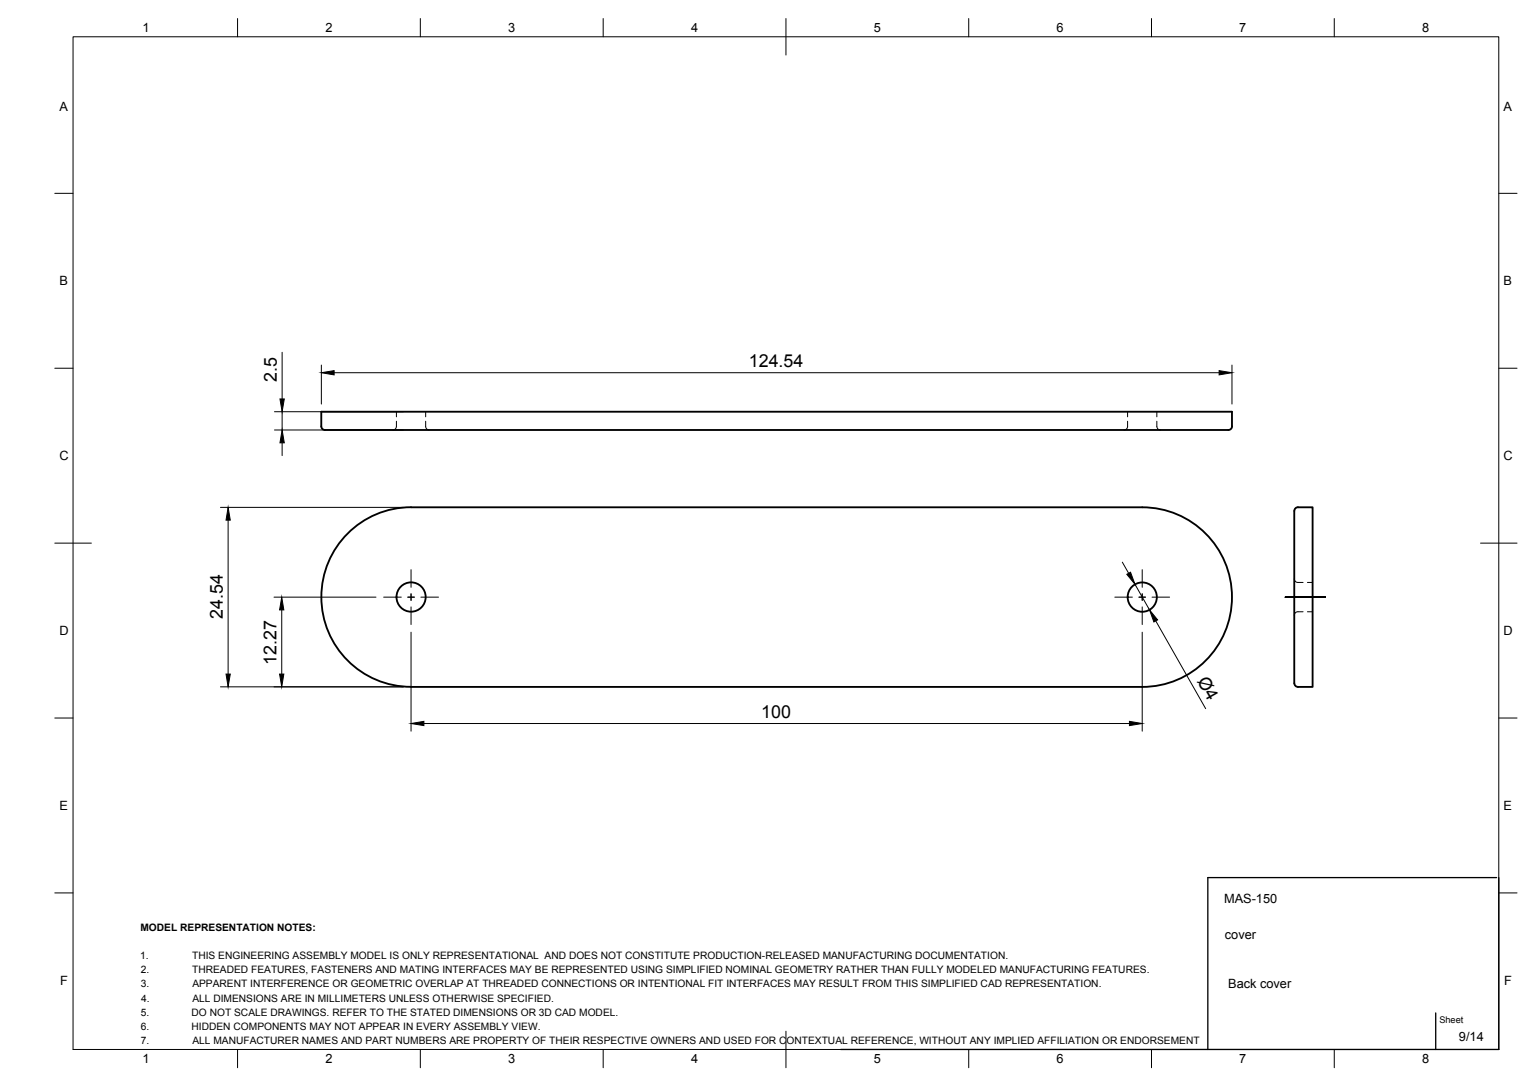
ISO-10303-21;
HEADER;
/* Generated by software containing ST-Developer
 * from STEP Tools, Inc. (www.steptools.com) 
 */

FILE_DESCRIPTION(
/* description */ ('STEP AP203'),
/* implementation_level */ '2;1');

FILE_NAME(
/* name */ 'Back cover.step',
/* time_stamp */ '2026-11-08T21:40:52-08:00',
/* author */ (''),
/* organization */ (''),
/* preprocessor_version */ 'ST-DEVELOPER v20.2',
/* originating_system */ 'Autodesk Translation Framework v15.17.0.0',
/* authorisation */ '');

FILE_SCHEMA (('AUTOMOTIVE_DESIGN { 1 0 10303 214 3 1 1 }'));
ENDSEC;

DATA;
#10=MECHANICAL_DESIGN_GEOMETRIC_PRESENTATION_REPRESENTATION('',(#191),#12137);
#169=SHAPE_REPRESENTATION_RELATIONSHIP('SRR','None',#12193,#180);
#180=ADVANCED_BREP_SHAPE_REPRESENTATION('',(#202),#12134);
#191=STYLED_ITEM('',(#12253),#202);
#202=MANIFOLD_SOLID_BREP('Body1',#1836);
#223=FACE_BOUND('',#704,.T.);
#224=FACE_BOUND('',#705,.T.);
#225=FACE_BOUND('',#707,.T.);
#226=FACE_BOUND('',#708,.T.);
#265=PLANE('',#2095);
#266=PLANE('',#2098);
#267=PLANE('',#2103);
#268=PLANE('',#2106);
#346=LINE('',#11987,#440);
#347=LINE('',#11991,#441);
#348=LINE('',#11998,#442);
#349=LINE('',#12001,#443);
#350=LINE('',#12007,#444);
#351=LINE('',#12010,#445);
#352=LINE('',#12013,#446);
#353=LINE('',#12016,#447);
#354=LINE('',#12019,#448);
#355=LINE('',#12020,#449);
#356=LINE('',#12023,#450);
#357=LINE('',#12026,#451);
#440=VECTOR('',#2492,2.);
#441=VECTOR('',#2497,2.);
#442=VECTOR('',#2504,1000.);
#443=VECTOR('',#2507,1000.);
#444=VECTOR('',#2512,1000.);
#445=VECTOR('',#2515,1000.);
#446=VECTOR('',#2518,1000.);
#447=VECTOR('',#2521,1000.);
#448=VECTOR('',#2524,1000.);
#449=VECTOR('',#2525,1000.);
#450=VECTOR('',#2528,1000.);
#451=VECTOR('',#2533,1000.);
#478=CYLINDRICAL_SURFACE('',#2091,2.);
#479=CYLINDRICAL_SURFACE('',#2093,2.);
#480=CYLINDRICAL_SURFACE('',#2101,12.2723008899906);
#481=CYLINDRICAL_SURFACE('',#2104,12.2723008899906);
#482=CYLINDRICAL_SURFACE('',#2107,0.5);
#483=CYLINDRICAL_SURFACE('',#2114,0.5);
#571=FACE_OUTER_BOUND('',#699,.T.);
#572=FACE_OUTER_BOUND('',#700,.T.);
#573=FACE_OUTER_BOUND('',#701,.T.);
#574=FACE_OUTER_BOUND('',#702,.T.);
#575=FACE_OUTER_BOUND('',#703,.T.);
#576=FACE_OUTER_BOUND('',#706,.T.);
#577=FACE_OUTER_BOUND('',#709,.T.);
#578=FACE_OUTER_BOUND('',#710,.T.);
#579=FACE_OUTER_BOUND('',#711,.T.);
#580=FACE_OUTER_BOUND('',#712,.T.);
#581=FACE_OUTER_BOUND('',#713,.T.);
#582=FACE_OUTER_BOUND('',#714,.T.);
#583=FACE_OUTER_BOUND('',#715,.T.);
#584=FACE_OUTER_BOUND('',#716,.T.);
#699=EDGE_LOOP('',(#1587,#1588,#1589,#1590,#1591));
#700=EDGE_LOOP('',(#1592,#1593,#1594,#1595,#1596));
#701=EDGE_LOOP('',(#1597,#1598,#1599,#1600,#1601));
#702=EDGE_LOOP('',(#1602,#1603,#1604,#1605,#1606));
#703=EDGE_LOOP('',(#1607,#1608,#1609,#1610));
#704=EDGE_LOOP('',(#1611));
#705=EDGE_LOOP('',(#1612));
#706=EDGE_LOOP('',(#1613,#1614,#1615,#1616));
#707=EDGE_LOOP('',(#1617));
#708=EDGE_LOOP('',(#1618));
#709=EDGE_LOOP('',(#1619,#1620,#1621,#1622));
#710=EDGE_LOOP('',(#1623,#1624,#1625,#1626));
#711=EDGE_LOOP('',(#1627,#1628,#1629,#1630));
#712=EDGE_LOOP('',(#1631,#1632,#1633,#1634));
#713=EDGE_LOOP('',(#1635,#1636,#1637,#1638));
#714=EDGE_LOOP('',(#1639,#1640,#1641,#1642));
#715=EDGE_LOOP('',(#1643,#1644,#1645,#1646));
#716=EDGE_LOOP('',(#1647,#1648,#1649,#1650));
#788=CIRCLE('',#2082,2.);
#789=CIRCLE('',#2083,2.);
#790=CIRCLE('',#2084,0.5);
#791=CIRCLE('',#2085,2.5);
#792=CIRCLE('',#2087,2.);
#793=CIRCLE('',#2088,2.);
#794=CIRCLE('',#2089,0.5);
#795=CIRCLE('',#2090,2.5);
#796=CIRCLE('',#2092,2.);
#797=CIRCLE('',#2094,2.);
#798=CIRCLE('',#2096,11.7723008899906);
#799=CIRCLE('',#2097,11.7723008899906);
#800=CIRCLE('',#2099,12.2723008899906);
#801=CIRCLE('',#2100,12.2723008899906);
#802=CIRCLE('',#2102,12.2723008899906);
#803=CIRCLE('',#2105,12.2723008899906);
#804=CIRCLE('',#2108,0.5);
#805=CIRCLE('',#2109,0.5);
#806=CIRCLE('',#2111,0.5);
#807=CIRCLE('',#2113,0.5);
#943=VERTEX_POINT('',#11970);
#944=VERTEX_POINT('',#11971);
#945=VERTEX_POINT('',#11974);
#946=VERTEX_POINT('',#11978);
#947=VERTEX_POINT('',#11979);
#948=VERTEX_POINT('',#11982);
#949=VERTEX_POINT('',#11986);
#950=VERTEX_POINT('',#11990);
#951=VERTEX_POINT('',#11994);
#952=VERTEX_POINT('',#11995);
#953=VERTEX_POINT('',#11997);
#954=VERTEX_POINT('',#11999);
#955=VERTEX_POINT('',#12003);
#956=VERTEX_POINT('',#12004);
#957=VERTEX_POINT('',#12006);
#958=VERTEX_POINT('',#12008);
#959=VERTEX_POINT('',#12012);
#960=VERTEX_POINT('',#12014);
#961=VERTEX_POINT('',#12018);
#962=VERTEX_POINT('',#12022);
#1163=EDGE_CURVE('',#943,#944,#788,.T.);
#1164=EDGE_CURVE('',#944,#943,#789,.T.);
#1165=EDGE_CURVE('',#944,#945,#790,.T.);
#1166=EDGE_CURVE('',#945,#945,#791,.T.);
#1167=EDGE_CURVE('',#946,#947,#792,.T.);
#1168=EDGE_CURVE('',#947,#946,#793,.T.);
#1169=EDGE_CURVE('',#947,#948,#794,.T.);
#1170=EDGE_CURVE('',#948,#948,#795,.T.);
#1171=EDGE_CURVE('',#946,#949,#346,.T.);
#1172=EDGE_CURVE('',#949,#949,#796,.T.);
#1173=EDGE_CURVE('',#943,#950,#347,.T.);
#1174=EDGE_CURVE('',#950,#950,#797,.T.);
#1175=EDGE_CURVE('',#951,#952,#798,.T.);
#1176=EDGE_CURVE('',#952,#953,#348,.T.);
#1177=EDGE_CURVE('',#953,#954,#799,.T.);
#1178=EDGE_CURVE('',#954,#951,#349,.T.);
#1179=EDGE_CURVE('',#955,#956,#800,.T.);
#1180=EDGE_CURVE('',#957,#955,#350,.T.);
#1181=EDGE_CURVE('',#958,#957,#801,.T.);
#1182=EDGE_CURVE('',#956,#958,#351,.T.);
#1183=EDGE_CURVE('',#959,#956,#352,.T.);
#1184=EDGE_CURVE('',#959,#960,#802,.T.);
#1185=EDGE_CURVE('',#960,#955,#353,.T.);
#1186=EDGE_CURVE('',#961,#958,#354,.T.);
#1187=EDGE_CURVE('',#961,#959,#355,.T.);
#1188=EDGE_CURVE('',#962,#957,#356,.T.);
#1189=EDGE_CURVE('',#962,#961,#803,.T.);
#1190=EDGE_CURVE('',#960,#962,#357,.T.);
#1191=EDGE_CURVE('',#959,#954,#804,.T.);
#1192=EDGE_CURVE('',#951,#961,#805,.T.);
#1193=EDGE_CURVE('',#952,#962,#806,.T.);
#1194=EDGE_CURVE('',#960,#953,#807,.T.);
#1587=ORIENTED_EDGE('',*,*,#1163,.F.);
#1588=ORIENTED_EDGE('',*,*,#1164,.F.);
#1589=ORIENTED_EDGE('',*,*,#1165,.T.);
#1590=ORIENTED_EDGE('',*,*,#1166,.F.);
#1591=ORIENTED_EDGE('',*,*,#1165,.F.);
#1592=ORIENTED_EDGE('',*,*,#1167,.F.);
#1593=ORIENTED_EDGE('',*,*,#1168,.F.);
#1594=ORIENTED_EDGE('',*,*,#1169,.T.);
#1595=ORIENTED_EDGE('',*,*,#1170,.F.);
#1596=ORIENTED_EDGE('',*,*,#1169,.F.);
#1597=ORIENTED_EDGE('',*,*,#1167,.T.);
#1598=ORIENTED_EDGE('',*,*,#1168,.T.);
#1599=ORIENTED_EDGE('',*,*,#1171,.T.);
#1600=ORIENTED_EDGE('',*,*,#1172,.F.);
#1601=ORIENTED_EDGE('',*,*,#1171,.F.);
#1602=ORIENTED_EDGE('',*,*,#1163,.T.);
#1603=ORIENTED_EDGE('',*,*,#1164,.T.);
#1604=ORIENTED_EDGE('',*,*,#1173,.T.);
#1605=ORIENTED_EDGE('',*,*,#1174,.F.);
#1606=ORIENTED_EDGE('',*,*,#1173,.F.);
#1607=ORIENTED_EDGE('',*,*,#1175,.T.);
#1608=ORIENTED_EDGE('',*,*,#1176,.T.);
#1609=ORIENTED_EDGE('',*,*,#1177,.T.);
#1610=ORIENTED_EDGE('',*,*,#1178,.T.);
#1611=ORIENTED_EDGE('',*,*,#1166,.T.);
#1612=ORIENTED_EDGE('',*,*,#1170,.T.);
#1613=ORIENTED_EDGE('',*,*,#1179,.F.);
#1614=ORIENTED_EDGE('',*,*,#1180,.F.);
#1615=ORIENTED_EDGE('',*,*,#1181,.F.);
#1616=ORIENTED_EDGE('',*,*,#1182,.F.);
#1617=ORIENTED_EDGE('',*,*,#1174,.T.);
#1618=ORIENTED_EDGE('',*,*,#1172,.T.);
#1619=ORIENTED_EDGE('',*,*,#1183,.F.);
#1620=ORIENTED_EDGE('',*,*,#1184,.T.);
#1621=ORIENTED_EDGE('',*,*,#1185,.T.);
#1622=ORIENTED_EDGE('',*,*,#1179,.T.);
#1623=ORIENTED_EDGE('',*,*,#1186,.F.);
#1624=ORIENTED_EDGE('',*,*,#1187,.T.);
#1625=ORIENTED_EDGE('',*,*,#1183,.T.);
#1626=ORIENTED_EDGE('',*,*,#1182,.T.);
#1627=ORIENTED_EDGE('',*,*,#1188,.F.);
#1628=ORIENTED_EDGE('',*,*,#1189,.T.);
#1629=ORIENTED_EDGE('',*,*,#1186,.T.);
#1630=ORIENTED_EDGE('',*,*,#1181,.T.);
#1631=ORIENTED_EDGE('',*,*,#1185,.F.);
#1632=ORIENTED_EDGE('',*,*,#1190,.T.);
#1633=ORIENTED_EDGE('',*,*,#1188,.T.);
#1634=ORIENTED_EDGE('',*,*,#1180,.T.);
#1635=ORIENTED_EDGE('',*,*,#1191,.F.);
#1636=ORIENTED_EDGE('',*,*,#1187,.F.);
#1637=ORIENTED_EDGE('',*,*,#1192,.F.);
#1638=ORIENTED_EDGE('',*,*,#1178,.F.);
#1639=ORIENTED_EDGE('',*,*,#1192,.T.);
#1640=ORIENTED_EDGE('',*,*,#1189,.F.);
#1641=ORIENTED_EDGE('',*,*,#1193,.F.);
#1642=ORIENTED_EDGE('',*,*,#1175,.F.);
#1643=ORIENTED_EDGE('',*,*,#1191,.T.);
#1644=ORIENTED_EDGE('',*,*,#1177,.F.);
#1645=ORIENTED_EDGE('',*,*,#1194,.F.);
#1646=ORIENTED_EDGE('',*,*,#1184,.F.);
#1647=ORIENTED_EDGE('',*,*,#1193,.T.);
#1648=ORIENTED_EDGE('',*,*,#1190,.F.);
#1649=ORIENTED_EDGE('',*,*,#1194,.T.);
#1650=ORIENTED_EDGE('',*,*,#1176,.F.);
#1712=TOROIDAL_SURFACE('',#2081,2.5,0.5);
#1713=TOROIDAL_SURFACE('',#2086,2.5,0.5);
#1714=TOROIDAL_SURFACE('',#2110,11.7723008899906,0.5);
#1715=TOROIDAL_SURFACE('',#2112,11.7723008899906,0.5);
#1799=ADVANCED_FACE('',(#571),#1712,.T.);
#1800=ADVANCED_FACE('',(#572),#1713,.T.);
#1801=ADVANCED_FACE('',(#573),#478,.F.);
#1802=ADVANCED_FACE('',(#574),#479,.F.);
#1803=ADVANCED_FACE('',(#575,#223,#224),#265,.T.);
#1804=ADVANCED_FACE('',(#576,#225,#226),#266,.F.);
#1805=ADVANCED_FACE('',(#577),#480,.T.);
#1806=ADVANCED_FACE('',(#578),#267,.F.);
#1807=ADVANCED_FACE('',(#579),#481,.T.);
#1808=ADVANCED_FACE('',(#580),#268,.F.);
#1809=ADVANCED_FACE('',(#581),#482,.T.);
#1810=ADVANCED_FACE('',(#582),#1714,.T.);
#1811=ADVANCED_FACE('',(#583),#1715,.T.);
#1812=ADVANCED_FACE('',(#584),#483,.T.);
#1836=CLOSED_SHELL('',(#1799,#1800,#1801,#1802,#1803,#1804,#1805,#1806,
#1807,#1808,#1809,#1810,#1811,#1812));
#2080=AXIS2_PLACEMENT_3D('',#11968,#2468,#2469);
#2081=AXIS2_PLACEMENT_3D('',#11969,#2470,#2471);
#2082=AXIS2_PLACEMENT_3D('',#11972,#2472,#2473);
#2083=AXIS2_PLACEMENT_3D('',#11973,#2474,#2475);
#2084=AXIS2_PLACEMENT_3D('',#11975,#2476,#2477);
#2085=AXIS2_PLACEMENT_3D('',#11976,#2478,#2479);
#2086=AXIS2_PLACEMENT_3D('',#11977,#2480,#2481);
#2087=AXIS2_PLACEMENT_3D('',#11980,#2482,#2483);
#2088=AXIS2_PLACEMENT_3D('',#11981,#2484,#2485);
#2089=AXIS2_PLACEMENT_3D('',#11983,#2486,#2487);
#2090=AXIS2_PLACEMENT_3D('',#11984,#2488,#2489);
#2091=AXIS2_PLACEMENT_3D('',#11985,#2490,#2491);
#2092=AXIS2_PLACEMENT_3D('',#11988,#2493,#2494);
#2093=AXIS2_PLACEMENT_3D('',#11989,#2495,#2496);
#2094=AXIS2_PLACEMENT_3D('',#11992,#2498,#2499);
#2095=AXIS2_PLACEMENT_3D('',#11993,#2500,#2501);
#2096=AXIS2_PLACEMENT_3D('',#11996,#2502,#2503);
#2097=AXIS2_PLACEMENT_3D('',#12000,#2505,#2506);
#2098=AXIS2_PLACEMENT_3D('',#12002,#2508,#2509);
#2099=AXIS2_PLACEMENT_3D('',#12005,#2510,#2511);
#2100=AXIS2_PLACEMENT_3D('',#12009,#2513,#2514);
#2101=AXIS2_PLACEMENT_3D('',#12011,#2516,#2517);
#2102=AXIS2_PLACEMENT_3D('',#12015,#2519,#2520);
#2103=AXIS2_PLACEMENT_3D('',#12017,#2522,#2523);
#2104=AXIS2_PLACEMENT_3D('',#12021,#2526,#2527);
#2105=AXIS2_PLACEMENT_3D('',#12024,#2529,#2530);
#2106=AXIS2_PLACEMENT_3D('',#12025,#2531,#2532);
#2107=AXIS2_PLACEMENT_3D('',#12027,#2534,#2535);
#2108=AXIS2_PLACEMENT_3D('',#12028,#2536,#2537);
#2109=AXIS2_PLACEMENT_3D('',#12029,#2538,#2539);
#2110=AXIS2_PLACEMENT_3D('',#12030,#2540,#2541);
#2111=AXIS2_PLACEMENT_3D('',#12031,#2542,#2543);
#2112=AXIS2_PLACEMENT_3D('',#12032,#2544,#2545);
#2113=AXIS2_PLACEMENT_3D('',#12033,#2546,#2547);
#2114=AXIS2_PLACEMENT_3D('',#12034,#2548,#2549);
#2468=DIRECTION('axis',(0.,0.,1.));
#2469=DIRECTION('refdir',(1.,0.,0.));
#2470=DIRECTION('center_axis',(0.,1.,0.));
#2471=DIRECTION('ref_axis',(0.,0.,1.));
#2472=DIRECTION('center_axis',(0.,1.,0.));
#2473=DIRECTION('ref_axis',(0.,0.,1.));
#2474=DIRECTION('center_axis',(0.,1.,0.));
#2475=DIRECTION('ref_axis',(0.,0.,1.));
#2476=DIRECTION('center_axis',(-1.,0.,0.));
#2477=DIRECTION('ref_axis',(0.,0.,-1.));
#2478=DIRECTION('center_axis',(0.,-1.,0.));
#2479=DIRECTION('ref_axis',(0.,0.,1.));
#2480=DIRECTION('center_axis',(0.,1.,0.));
#2481=DIRECTION('ref_axis',(0.,0.,1.));
#2482=DIRECTION('center_axis',(0.,1.,0.));
#2483=DIRECTION('ref_axis',(0.,0.,1.));
#2484=DIRECTION('center_axis',(0.,1.,0.));
#2485=DIRECTION('ref_axis',(0.,0.,1.));
#2486=DIRECTION('center_axis',(-1.,0.,0.));
#2487=DIRECTION('ref_axis',(0.,0.,-1.));
#2488=DIRECTION('center_axis',(0.,-1.,0.));
#2489=DIRECTION('ref_axis',(0.,0.,1.));
#2490=DIRECTION('center_axis',(0.,-1.,0.));
#2491=DIRECTION('ref_axis',(0.,0.,-1.));
#2492=DIRECTION('',(0.,-1.,0.));
#2493=DIRECTION('center_axis',(0.,1.,0.));
#2494=DIRECTION('ref_axis',(0.,0.,1.));
#2495=DIRECTION('center_axis',(0.,-1.,0.));
#2496=DIRECTION('ref_axis',(0.,0.,-1.));
#2497=DIRECTION('',(0.,-1.,0.));
#2498=DIRECTION('center_axis',(0.,1.,0.));
#2499=DIRECTION('ref_axis',(0.,0.,1.));
#2500=DIRECTION('center_axis',(0.,1.,0.));
#2501=DIRECTION('ref_axis',(0.,0.,1.));
#2502=DIRECTION('center_axis',(0.,1.,0.));
#2503=DIRECTION('ref_axis',(0.,0.,1.));
#2504=DIRECTION('',(1.,0.,-7.77156117237611E-15));
#2505=DIRECTION('center_axis',(0.,1.,0.));
#2506=DIRECTION('ref_axis',(0.,0.,1.));
#2507=DIRECTION('',(-1.,0.,7.77156117237609E-15));
#2508=DIRECTION('center_axis',(0.,1.,0.));
#2509=DIRECTION('ref_axis',(0.,0.,1.));
#2510=DIRECTION('center_axis',(0.,1.,0.));
#2511=DIRECTION('ref_axis',(0.,0.,1.));
#2512=DIRECTION('',(1.,0.,-7.77156117237611E-15));
#2513=DIRECTION('center_axis',(0.,1.,0.));
#2514=DIRECTION('ref_axis',(0.,0.,1.));
#2515=DIRECTION('',(-1.,0.,7.77156117237609E-15));
#2516=DIRECTION('center_axis',(0.,-1.,0.));
#2517=DIRECTION('ref_axis',(0.,0.,-1.));
#2518=DIRECTION('',(0.,-1.,0.));
#2519=DIRECTION('center_axis',(0.,-1.,0.));
#2520=DIRECTION('ref_axis',(0.,0.,1.));
#2521=DIRECTION('',(0.,-1.,0.));
#2522=DIRECTION('center_axis',(7.77156117237609E-15,0.,1.));
#2523=DIRECTION('ref_axis',(1.,0.,-7.77156117237609E-15));
#2524=DIRECTION('',(0.,-1.,0.));
#2525=DIRECTION('',(1.,0.,-7.77156117237609E-15));
#2526=DIRECTION('center_axis',(0.,-1.,0.));
#2527=DIRECTION('ref_axis',(0.,0.,-1.));
#2528=DIRECTION('',(0.,-1.,0.));
#2529=DIRECTION('center_axis',(0.,-1.,0.));
#2530=DIRECTION('ref_axis',(0.,0.,1.));
#2531=DIRECTION('center_axis',(-7.77156117237611E-15,0.,-1.));
#2532=DIRECTION('ref_axis',(-1.,0.,7.77156117237611E-15));
#2533=DIRECTION('',(-1.,0.,7.77156117237611E-15));
#2534=DIRECTION('center_axis',(1.,0.,-7.77156117237609E-15));
#2535=DIRECTION('ref_axis',(-7.77156117237609E-15,0.,-1.));
#2536=DIRECTION('center_axis',(1.,0.,-6.93889390390722E-15));
#2537=DIRECTION('ref_axis',(-6.93889390390722E-15,0.,-1.));
#2538=DIRECTION('center_axis',(-1.,0.,0.));
#2539=DIRECTION('ref_axis',(0.,0.,1.));
#2540=DIRECTION('center_axis',(0.,1.,0.));
#2541=DIRECTION('ref_axis',(0.,0.,1.));
#2542=DIRECTION('center_axis',(1.,0.,0.));
#2543=DIRECTION('ref_axis',(0.,0.,-1.));
#2544=DIRECTION('center_axis',(0.,1.,0.));
#2545=DIRECTION('ref_axis',(0.,0.,1.));
#2546=DIRECTION('center_axis',(-1.,-6.93889390390723E-15,0.));
#2547=DIRECTION('ref_axis',(6.93889390390723E-15,-1.,0.));
#2548=DIRECTION('center_axis',(-1.,0.,7.77156117237611E-15));
#2549=DIRECTION('ref_axis',(7.77156117237611E-15,0.,1.));
#11968=CARTESIAN_POINT('',(0.,0.,0.));
#11969=CARTESIAN_POINT('Origin',(-83.4892602927113,2.,28.6344795489034));
#11970=CARTESIAN_POINT('',(-83.4892602927113,2.,30.6344795489034));
#11971=CARTESIAN_POINT('',(-83.4892602927113,2.,26.6344795489034));
#11972=CARTESIAN_POINT('Origin',(-83.4892602927113,2.,28.6344795489034));
#11973=CARTESIAN_POINT('Origin',(-83.4892602927113,2.,28.6344795489034));
#11974=CARTESIAN_POINT('',(-83.4892602927113,2.5,26.1344795489034));
#11975=CARTESIAN_POINT('Origin',(-83.4892602927113,2.,26.1344795489034));
#11976=CARTESIAN_POINT('Origin',(-83.4892602927113,2.5,28.6344795489034));
#11977=CARTESIAN_POINT('Origin',(16.5107397072887,2.,28.6344795489026));
#11978=CARTESIAN_POINT('',(16.5107397072887,2.,30.6344795489026));
#11979=CARTESIAN_POINT('',(16.5107397072887,2.,26.6344795489026));
#11980=CARTESIAN_POINT('Origin',(16.5107397072887,2.,28.6344795489026));
#11981=CARTESIAN_POINT('Origin',(16.5107397072887,2.,28.6344795489026));
#11982=CARTESIAN_POINT('',(16.5107397072887,2.5,26.1344795489026));
#11983=CARTESIAN_POINT('Origin',(16.5107397072887,2.,26.1344795489026));
#11984=CARTESIAN_POINT('Origin',(16.5107397072887,2.5,28.6344795489026));
#11985=CARTESIAN_POINT('Origin',(16.5107397072887,2.5,28.6344795489026));
#11986=CARTESIAN_POINT('',(16.5107397072887,0.,30.6344795489026));
#11987=CARTESIAN_POINT('',(16.5107397072887,2.5,30.6344795489026));
#11988=CARTESIAN_POINT('Origin',(16.5107397072887,0.,28.6344795489026));
#11989=CARTESIAN_POINT('Origin',(-83.4892602927113,2.5,28.6344795489034));
#11990=CARTESIAN_POINT('',(-83.4892602927113,0.,30.6344795489034));
#11991=CARTESIAN_POINT('',(-83.4892602927113,2.5,30.6344795489034));
#11992=CARTESIAN_POINT('Origin',(-83.4892602927113,0.,28.6344795489034));
#11993=CARTESIAN_POINT('Origin',(16.5107397072887,2.5,28.6344795489026));
#11994=CARTESIAN_POINT('',(-83.4892602927114,2.49999999999999,16.8621786589128));
#11995=CARTESIAN_POINT('',(-83.4892602927112,2.5,40.406780438894));
#11996=CARTESIAN_POINT('Origin',(-83.4892602927113,2.5,28.6344795489034));
#11997=CARTESIAN_POINT('',(16.5107397072887,2.5,40.4067804388932));
#11998=CARTESIAN_POINT('',(16.5107397072887,2.5,40.4067804388932));
#11999=CARTESIAN_POINT('',(16.5107397072887,2.49999999999999,16.862178658912));
#12000=CARTESIAN_POINT('Origin',(16.5107397072887,2.5,28.6344795489026));
#12001=CARTESIAN_POINT('',(-83.4892602927114,2.49999999999999,16.8621786589128));
#12002=CARTESIAN_POINT('Origin',(16.5107397072887,0.,28.6344795489026));
#12003=CARTESIAN_POINT('',(16.5107397072887,-1.38777878078145E-14,40.9067804388932));
#12004=CARTESIAN_POINT('',(16.5107397072887,-1.38777878078145E-14,16.362178658912));
#12005=CARTESIAN_POINT('Origin',(16.5107397072887,0.,28.6344795489026));
#12006=CARTESIAN_POINT('',(-83.4892602927112,-1.38777878078145E-14,40.9067804388939));
#12007=CARTESIAN_POINT('',(16.5107397072887,-1.38777878078145E-14,40.9067804388932));
#12008=CARTESIAN_POINT('',(-83.4892602927114,-1.38777878078145E-14,16.3621786589128));
#12009=CARTESIAN_POINT('Origin',(-83.4892602927113,0.,28.6344795489034));
#12010=CARTESIAN_POINT('',(16.5107397072887,-1.38777878078145E-14,16.362178658912));
#12011=CARTESIAN_POINT('Origin',(16.5107397072887,2.5,28.6344795489026));
#12012=CARTESIAN_POINT('',(16.5107397072887,2.,16.362178658912));
#12013=CARTESIAN_POINT('',(16.5107397072887,2.5,16.362178658912));
#12014=CARTESIAN_POINT('',(16.5107397072887,2.,40.9067804388932));
#12015=CARTESIAN_POINT('Origin',(16.5107397072887,2.,28.6344795489026));
#12016=CARTESIAN_POINT('',(16.5107397072887,2.5,40.9067804388932));
#12017=CARTESIAN_POINT('Origin',(16.5107397072887,2.5,16.362178658912));
#12018=CARTESIAN_POINT('',(-83.4892602927114,2.,16.3621786589128));
#12019=CARTESIAN_POINT('',(-83.4892602927114,2.5,16.3621786589128));
#12020=CARTESIAN_POINT('',(16.5107397072887,2.,16.362178658912));
#12021=CARTESIAN_POINT('Origin',(-83.4892602927113,2.5,28.6344795489034));
#12022=CARTESIAN_POINT('',(-83.4892602927112,2.,40.9067804388939));
#12023=CARTESIAN_POINT('',(-83.4892602927112,2.5,40.906780438894));
#12024=CARTESIAN_POINT('Origin',(-83.4892602927113,2.,28.6344795489034));
#12025=CARTESIAN_POINT('Origin',(16.5107397072887,2.5,40.9067804388932));
#12026=CARTESIAN_POINT('',(-83.4892602927112,2.,40.9067804388939));
#12027=CARTESIAN_POINT('Origin',(16.5107397072886,2.,16.862178658912));
#12028=CARTESIAN_POINT('Origin',(16.5107397072887,2.,16.862178658912));
#12029=CARTESIAN_POINT('Origin',(-83.4892602927114,2.,16.8621786589128));
#12030=CARTESIAN_POINT('Origin',(-83.4892602927113,2.,28.6344795489034));
#12031=CARTESIAN_POINT('Origin',(-83.4892602927112,2.,40.4067804388939));
#12032=CARTESIAN_POINT('Origin',(16.5107397072887,2.,28.6344795489026));
#12033=CARTESIAN_POINT('Origin',(16.5107397072887,2.,40.4067804388932));
#12034=CARTESIAN_POINT('Origin',(16.5107397072888,2.,40.4067804388932));
#12120=UNCERTAINTY_MEASURE_WITH_UNIT(LENGTH_MEASURE(0.01),#12138,
'DISTANCE_ACCURACY_VALUE',
'Maximum model space distance between geometric entities at asserted c
onnectivities');
#12123=UNCERTAINTY_MEASURE_WITH_UNIT(LENGTH_MEASURE(0.01),#12138,
'DISTANCE_ACCURACY_VALUE',
'Maximum model space distance between geometric entities at asserted c
onnectivities');
#12134=(
GEOMETRIC_REPRESENTATION_CONTEXT(3)
GLOBAL_UNCERTAINTY_ASSIGNED_CONTEXT((#12120))
GLOBAL_UNIT_ASSIGNED_CONTEXT((#12138,#12140,#12141))
REPRESENTATION_CONTEXT('','3D')
);
#12137=(
GEOMETRIC_REPRESENTATION_CONTEXT(3)
GLOBAL_UNCERTAINTY_ASSIGNED_CONTEXT((#12123))
GLOBAL_UNIT_ASSIGNED_CONTEXT((#12138,#12140,#12141))
REPRESENTATION_CONTEXT('','3D')
);
#12138=(
LENGTH_UNIT()
NAMED_UNIT(*)
SI_UNIT(.MILLI.,.METRE.)
);
#12140=(
NAMED_UNIT(*)
PLANE_ANGLE_UNIT()
SI_UNIT($,.RADIAN.)
);
#12141=(
NAMED_UNIT(*)
SI_UNIT($,.STERADIAN.)
SOLID_ANGLE_UNIT()
);
#12152=SHAPE_DEFINITION_REPRESENTATION(#12168,#12193);
#12168=PRODUCT_DEFINITION_SHAPE('',$,#12207);
#12193=SHAPE_REPRESENTATION('',(#2080),#12134);
#12196=PRODUCT_DEFINITION_CONTEXT('part definition',#12237,'design');
#12207=PRODUCT_DEFINITION('cover','Back cover',#12220,#12196);
#12220=PRODUCT_DEFINITION_FORMATION('',$,#12249);
#12237=APPLICATION_CONTEXT(
'Core Data for Automotive Mechanical Design Process');
#12238=PRODUCT_CONTEXT('part definition',#12237,'mechanical');
#12249=PRODUCT('cover','Back cover',$,(#12238));
#12253=PRESENTATION_STYLE_ASSIGNMENT((#12255));
#12255=SURFACE_STYLE_USAGE(.BOTH.,#12257);
#12257=SURFACE_SIDE_STYLE('',(#12259));
#12259=SURFACE_STYLE_FILL_AREA(#12261);
#12261=FILL_AREA_STYLE('Opaque(23,69,131)',(#12263));
#12263=FILL_AREA_STYLE_COLOUR('Opaque(23,69,131)',#12265);
#12265=COLOUR_RGB('Opaque(23,69,131)',0.0901960784313725,0.270588235294118,
0.513725490196078);
ENDSEC;
END-ISO-10303-21;
